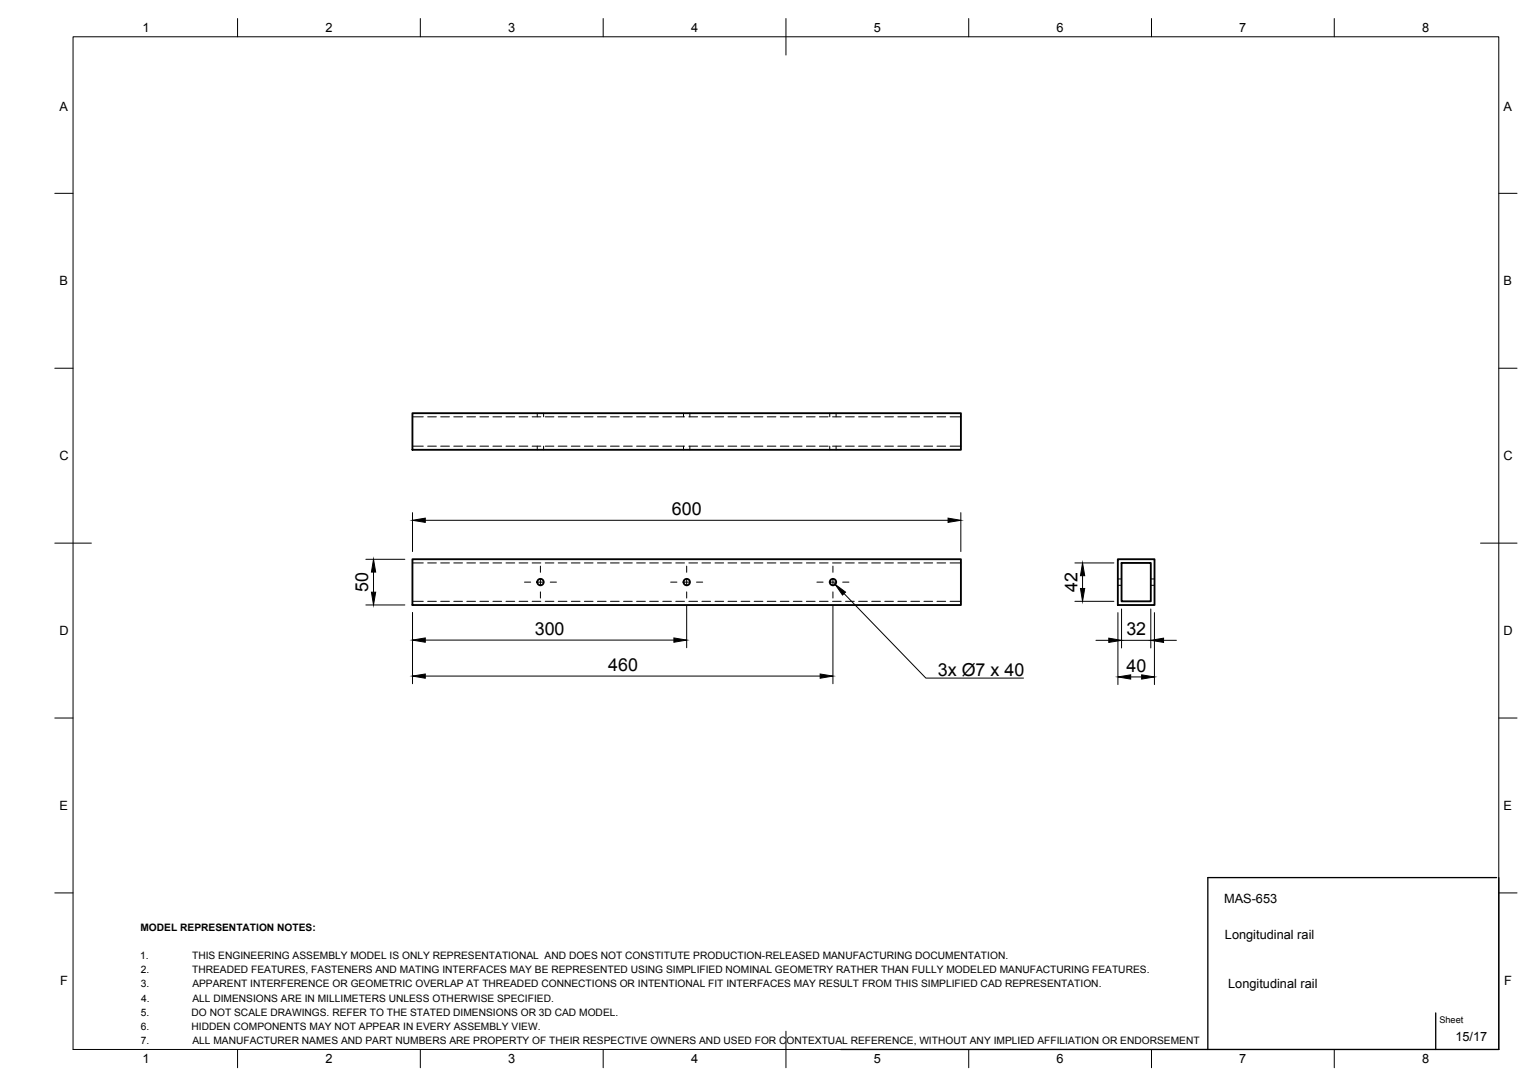
ISO-10303-21;
HEADER;
/* Generated by software containing ST-Developer
 * from STEP Tools, Inc. (www.steptools.com) 
 */

FILE_DESCRIPTION(
/* description */ ('Independent compact industrial fixture table, bolted aluminum worktop
 on connected adjustable support base. Whole-mm nominal dimensions. No
 load rating assigned.'),
/* implementation_level */ '2;1');

FILE_NAME(
/* name */ 'Longitudinal rail.step',
/* time_stamp */ '2026-11-07T17:47:58-08:00',
/* author */ (''),
/* organization */ (''),
/* preprocessor_version */ 'ST-DEVELOPER v20.2',
/* originating_system */ 'Autodesk Translation Framework v15.17.0.0',
/* authorisation */ '');

FILE_SCHEMA (('AUTOMOTIVE_DESIGN { 1 0 10303 214 3 1 1 }'));
ENDSEC;

DATA;
#10=MECHANICAL_DESIGN_GEOMETRIC_PRESENTATION_REPRESENTATION('',(#2250),#97475);
#2212=SHAPE_REPRESENTATION_RELATIONSHIP('SRR','None',#97605,#2231);
#2231=ADVANCED_BREP_SHAPE_REPRESENTATION('',(#2269),#97455);
#2250=STYLED_ITEM('',(#97718),#2269);
#2269=MANIFOLD_SOLID_BREP('Body1',#21811);
#2288=FACE_BOUND('',#3699,.T.);
#2289=FACE_BOUND('',#3700,.T.);
#2290=FACE_BOUND('',#3701,.T.);
#2291=FACE_BOUND('',#3704,.T.);
#2292=FACE_BOUND('',#3705,.T.);
#2293=FACE_BOUND('',#3706,.T.);
#2294=FACE_BOUND('',#3709,.T.);
#2295=FACE_BOUND('',#3710,.T.);
#2296=FACE_BOUND('',#3711,.T.);
#2297=FACE_BOUND('',#3714,.T.);
#2298=FACE_BOUND('',#3715,.T.);
#2299=FACE_BOUND('',#3716,.T.);
#2300=FACE_BOUND('',#3718,.T.);
#2301=FACE_BOUND('',#3720,.T.);
#2379=PLANE('',#22061);
#2380=PLANE('',#22062);
#2381=PLANE('',#22063);
#2382=PLANE('',#22064);
#2383=PLANE('',#22065);
#2384=PLANE('',#22066);
#2385=PLANE('',#22067);
#2386=PLANE('',#22068);
#2387=PLANE('',#22069);
#2388=PLANE('',#22070);
#2537=FACE_OUTER_BOUND('',#3691,.T.);
#2538=FACE_OUTER_BOUND('',#3692,.T.);
#2539=FACE_OUTER_BOUND('',#3693,.T.);
#2540=FACE_OUTER_BOUND('',#3694,.T.);
#2541=FACE_OUTER_BOUND('',#3695,.T.);
#2542=FACE_OUTER_BOUND('',#3696,.T.);
#2543=FACE_OUTER_BOUND('',#3697,.T.);
#2544=FACE_OUTER_BOUND('',#3698,.T.);
#2545=FACE_OUTER_BOUND('',#3702,.T.);
#2546=FACE_OUTER_BOUND('',#3703,.T.);
#2547=FACE_OUTER_BOUND('',#3707,.T.);
#2548=FACE_OUTER_BOUND('',#3708,.T.);
#2549=FACE_OUTER_BOUND('',#3712,.T.);
#2550=FACE_OUTER_BOUND('',#3713,.T.);
#2551=FACE_OUTER_BOUND('',#3717,.T.);
#2552=FACE_OUTER_BOUND('',#3719,.T.);
#3691=EDGE_LOOP('',(#13112,#13113,#13114,#13115));
#3692=EDGE_LOOP('',(#13116,#13117,#13118,#13119));
#3693=EDGE_LOOP('',(#13120,#13121,#13122,#13123));
#3694=EDGE_LOOP('',(#13124,#13125,#13126,#13127));
#3695=EDGE_LOOP('',(#13128,#13129,#13130,#13131));
#3696=EDGE_LOOP('',(#13132,#13133,#13134,#13135));
#3697=EDGE_LOOP('',(#13136,#13137,#13138,#13139));
#3698=EDGE_LOOP('',(#13140,#13141,#13142,#13143));
#3699=EDGE_LOOP('',(#13144));
#3700=EDGE_LOOP('',(#13145));
#3701=EDGE_LOOP('',(#13146));
#3702=EDGE_LOOP('',(#13147,#13148,#13149,#13150));
#3703=EDGE_LOOP('',(#13151,#13152,#13153,#13154));
#3704=EDGE_LOOP('',(#13155));
#3705=EDGE_LOOP('',(#13156));
#3706=EDGE_LOOP('',(#13157));
#3707=EDGE_LOOP('',(#13158,#13159,#13160,#13161));
#3708=EDGE_LOOP('',(#13162,#13163,#13164,#13165));
#3709=EDGE_LOOP('',(#13166));
#3710=EDGE_LOOP('',(#13167));
#3711=EDGE_LOOP('',(#13168));
#3712=EDGE_LOOP('',(#13169,#13170,#13171,#13172));
#3713=EDGE_LOOP('',(#13173,#13174,#13175,#13176));
#3714=EDGE_LOOP('',(#13177));
#3715=EDGE_LOOP('',(#13178));
#3716=EDGE_LOOP('',(#13179));
#3717=EDGE_LOOP('',(#13180,#13181,#13182,#13183));
#3718=EDGE_LOOP('',(#13184,#13185,#13186,#13187));
#3719=EDGE_LOOP('',(#13188,#13189,#13190,#13191));
#3720=EDGE_LOOP('',(#13192,#13193,#13194,#13195));
#4936=LINE('',#27647,#6150);
#4937=LINE('',#27653,#6151);
#4938=LINE('',#27659,#6152);
#4939=LINE('',#27665,#6153);
#4940=LINE('',#27671,#6154);
#4941=LINE('',#27677,#6155);
#4942=LINE('',#27682,#6156);
#4943=LINE('',#27684,#6157);
#4944=LINE('',#27686,#6158);
#4945=LINE('',#27687,#6159);
#4946=LINE('',#27690,#6160);
#4947=LINE('',#27692,#6161);
#4948=LINE('',#27693,#6162);
#4949=LINE('',#27696,#6163);
#4950=LINE('',#27698,#6164);
#4951=LINE('',#27699,#6165);
#4952=LINE('',#27701,#6166);
#4953=LINE('',#27702,#6167);
#4954=LINE('',#27706,#6168);
#4955=LINE('',#27708,#6169);
#4956=LINE('',#27710,#6170);
#4957=LINE('',#27711,#6171);
#4958=LINE('',#27714,#6172);
#4959=LINE('',#27716,#6173);
#4960=LINE('',#27717,#6174);
#4961=LINE('',#27720,#6175);
#4962=LINE('',#27722,#6176);
#4963=LINE('',#27723,#6177);
#4964=LINE('',#27725,#6178);
#4965=LINE('',#27726,#6179);
#6150=VECTOR('',#23512,3.5);
#6151=VECTOR('',#23519,3.5);
#6152=VECTOR('',#23526,3.5);
#6153=VECTOR('',#23533,3.5);
#6154=VECTOR('',#23540,3.5);
#6155=VECTOR('',#23547,3.5);
#6156=VECTOR('',#23552,10.);
#6157=VECTOR('',#23553,10.);
#6158=VECTOR('',#23554,10.);
#6159=VECTOR('',#23555,10.);
#6160=VECTOR('',#23558,10.);
#6161=VECTOR('',#23559,10.);
#6162=VECTOR('',#23560,10.);
#6163=VECTOR('',#23563,10.);
#6164=VECTOR('',#23564,10.);
#6165=VECTOR('',#23565,10.);
#6166=VECTOR('',#23568,10.);
#6167=VECTOR('',#23569,10.);
#6168=VECTOR('',#23572,10.);
#6169=VECTOR('',#23573,10.);
#6170=VECTOR('',#23574,10.);
#6171=VECTOR('',#23575,10.);
#6172=VECTOR('',#23578,10.);
#6173=VECTOR('',#23579,10.);
#6174=VECTOR('',#23580,10.);
#6175=VECTOR('',#23583,10.);
#6176=VECTOR('',#23584,10.);
#6177=VECTOR('',#23585,10.);
#6178=VECTOR('',#23588,10.);
#6179=VECTOR('',#23589,10.);
#7364=CIRCLE('',#22044,3.5);
#7365=CIRCLE('',#22045,3.5);
#7366=CIRCLE('',#22047,3.5);
#7367=CIRCLE('',#22048,3.5);
#7368=CIRCLE('',#22050,3.5);
#7369=CIRCLE('',#22051,3.5);
#7370=CIRCLE('',#22053,3.5);
#7371=CIRCLE('',#22054,3.5);
#7372=CIRCLE('',#22056,3.5);
#7373=CIRCLE('',#22057,3.5);
#7374=CIRCLE('',#22059,3.5);
#7375=CIRCLE('',#22060,3.5);
#7613=VERTEX_POINT('',#27644);
#7614=VERTEX_POINT('',#27646);
#7615=VERTEX_POINT('',#27650);
#7616=VERTEX_POINT('',#27652);
#7617=VERTEX_POINT('',#27656);
#7618=VERTEX_POINT('',#27658);
#7619=VERTEX_POINT('',#27662);
#7620=VERTEX_POINT('',#27664);
#7621=VERTEX_POINT('',#27668);
#7622=VERTEX_POINT('',#27670);
#7623=VERTEX_POINT('',#27674);
#7624=VERTEX_POINT('',#27676);
#7625=VERTEX_POINT('',#27680);
#7626=VERTEX_POINT('',#27681);
#7627=VERTEX_POINT('',#27683);
#7628=VERTEX_POINT('',#27685);
#7629=VERTEX_POINT('',#27689);
#7630=VERTEX_POINT('',#27691);
#7631=VERTEX_POINT('',#27695);
#7632=VERTEX_POINT('',#27697);
#7633=VERTEX_POINT('',#27704);
#7634=VERTEX_POINT('',#27705);
#7635=VERTEX_POINT('',#27707);
#7636=VERTEX_POINT('',#27709);
#7637=VERTEX_POINT('',#27713);
#7638=VERTEX_POINT('',#27715);
#7639=VERTEX_POINT('',#27719);
#7640=VERTEX_POINT('',#27721);
#9813=EDGE_CURVE('',#7613,#7613,#7364,.T.);
#9814=EDGE_CURVE('',#7613,#7614,#4936,.T.);
#9815=EDGE_CURVE('',#7614,#7614,#7365,.T.);
#9816=EDGE_CURVE('',#7615,#7615,#7366,.T.);
#9817=EDGE_CURVE('',#7615,#7616,#4937,.T.);
#9818=EDGE_CURVE('',#7616,#7616,#7367,.T.);
#9819=EDGE_CURVE('',#7617,#7617,#7368,.T.);
#9820=EDGE_CURVE('',#7617,#7618,#4938,.T.);
#9821=EDGE_CURVE('',#7618,#7618,#7369,.T.);
#9822=EDGE_CURVE('',#7619,#7619,#7370,.T.);
#9823=EDGE_CURVE('',#7619,#7620,#4939,.T.);
#9824=EDGE_CURVE('',#7620,#7620,#7371,.T.);
#9825=EDGE_CURVE('',#7621,#7621,#7372,.T.);
#9826=EDGE_CURVE('',#7621,#7622,#4940,.T.);
#9827=EDGE_CURVE('',#7622,#7622,#7373,.T.);
#9828=EDGE_CURVE('',#7623,#7623,#7374,.T.);
#9829=EDGE_CURVE('',#7623,#7624,#4941,.T.);
#9830=EDGE_CURVE('',#7624,#7624,#7375,.T.);
#9831=EDGE_CURVE('',#7625,#7626,#4942,.T.);
#9832=EDGE_CURVE('',#7626,#7627,#4943,.T.);
#9833=EDGE_CURVE('',#7628,#7627,#4944,.T.);
#9834=EDGE_CURVE('',#7625,#7628,#4945,.T.);
#9835=EDGE_CURVE('',#7629,#7625,#4946,.T.);
#9836=EDGE_CURVE('',#7630,#7628,#4947,.T.);
#9837=EDGE_CURVE('',#7629,#7630,#4948,.T.);
#9838=EDGE_CURVE('',#7631,#7629,#4949,.T.);
#9839=EDGE_CURVE('',#7632,#7630,#4950,.T.);
#9840=EDGE_CURVE('',#7631,#7632,#4951,.T.);
#9841=EDGE_CURVE('',#7626,#7631,#4952,.T.);
#9842=EDGE_CURVE('',#7627,#7632,#4953,.T.);
#9843=EDGE_CURVE('',#7633,#7634,#4954,.T.);
#9844=EDGE_CURVE('',#7634,#7635,#4955,.T.);
#9845=EDGE_CURVE('',#7636,#7635,#4956,.T.);
#9846=EDGE_CURVE('',#7633,#7636,#4957,.T.);
#9847=EDGE_CURVE('',#7637,#7633,#4958,.T.);
#9848=EDGE_CURVE('',#7638,#7636,#4959,.T.);
#9849=EDGE_CURVE('',#7637,#7638,#4960,.T.);
#9850=EDGE_CURVE('',#7639,#7637,#4961,.T.);
#9851=EDGE_CURVE('',#7640,#7638,#4962,.T.);
#9852=EDGE_CURVE('',#7639,#7640,#4963,.T.);
#9853=EDGE_CURVE('',#7634,#7639,#4964,.T.);
#9854=EDGE_CURVE('',#7635,#7640,#4965,.T.);
#13112=ORIENTED_EDGE('',*,*,#9813,.F.);
#13113=ORIENTED_EDGE('',*,*,#9814,.T.);
#13114=ORIENTED_EDGE('',*,*,#9815,.F.);
#13115=ORIENTED_EDGE('',*,*,#9814,.F.);
#13116=ORIENTED_EDGE('',*,*,#9816,.F.);
#13117=ORIENTED_EDGE('',*,*,#9817,.T.);
#13118=ORIENTED_EDGE('',*,*,#9818,.F.);
#13119=ORIENTED_EDGE('',*,*,#9817,.F.);
#13120=ORIENTED_EDGE('',*,*,#9819,.F.);
#13121=ORIENTED_EDGE('',*,*,#9820,.T.);
#13122=ORIENTED_EDGE('',*,*,#9821,.F.);
#13123=ORIENTED_EDGE('',*,*,#9820,.F.);
#13124=ORIENTED_EDGE('',*,*,#9822,.F.);
#13125=ORIENTED_EDGE('',*,*,#9823,.T.);
#13126=ORIENTED_EDGE('',*,*,#9824,.F.);
#13127=ORIENTED_EDGE('',*,*,#9823,.F.);
#13128=ORIENTED_EDGE('',*,*,#9825,.F.);
#13129=ORIENTED_EDGE('',*,*,#9826,.T.);
#13130=ORIENTED_EDGE('',*,*,#9827,.F.);
#13131=ORIENTED_EDGE('',*,*,#9826,.F.);
#13132=ORIENTED_EDGE('',*,*,#9828,.F.);
#13133=ORIENTED_EDGE('',*,*,#9829,.T.);
#13134=ORIENTED_EDGE('',*,*,#9830,.F.);
#13135=ORIENTED_EDGE('',*,*,#9829,.F.);
#13136=ORIENTED_EDGE('',*,*,#9831,.T.);
#13137=ORIENTED_EDGE('',*,*,#9832,.T.);
#13138=ORIENTED_EDGE('',*,*,#9833,.F.);
#13139=ORIENTED_EDGE('',*,*,#9834,.F.);
#13140=ORIENTED_EDGE('',*,*,#9835,.T.);
#13141=ORIENTED_EDGE('',*,*,#9834,.T.);
#13142=ORIENTED_EDGE('',*,*,#9836,.F.);
#13143=ORIENTED_EDGE('',*,*,#9837,.F.);
#13144=ORIENTED_EDGE('',*,*,#9818,.T.);
#13145=ORIENTED_EDGE('',*,*,#9824,.T.);
#13146=ORIENTED_EDGE('',*,*,#9830,.T.);
#13147=ORIENTED_EDGE('',*,*,#9838,.T.);
#13148=ORIENTED_EDGE('',*,*,#9837,.T.);
#13149=ORIENTED_EDGE('',*,*,#9839,.F.);
#13150=ORIENTED_EDGE('',*,*,#9840,.F.);
#13151=ORIENTED_EDGE('',*,*,#9841,.T.);
#13152=ORIENTED_EDGE('',*,*,#9840,.T.);
#13153=ORIENTED_EDGE('',*,*,#9842,.F.);
#13154=ORIENTED_EDGE('',*,*,#9832,.F.);
#13155=ORIENTED_EDGE('',*,*,#9813,.T.);
#13156=ORIENTED_EDGE('',*,*,#9819,.T.);
#13157=ORIENTED_EDGE('',*,*,#9825,.T.);
#13158=ORIENTED_EDGE('',*,*,#9843,.T.);
#13159=ORIENTED_EDGE('',*,*,#9844,.T.);
#13160=ORIENTED_EDGE('',*,*,#9845,.F.);
#13161=ORIENTED_EDGE('',*,*,#9846,.F.);
#13162=ORIENTED_EDGE('',*,*,#9847,.T.);
#13163=ORIENTED_EDGE('',*,*,#9846,.T.);
#13164=ORIENTED_EDGE('',*,*,#9848,.F.);
#13165=ORIENTED_EDGE('',*,*,#9849,.F.);
#13166=ORIENTED_EDGE('',*,*,#9816,.T.);
#13167=ORIENTED_EDGE('',*,*,#9822,.T.);
#13168=ORIENTED_EDGE('',*,*,#9828,.T.);
#13169=ORIENTED_EDGE('',*,*,#9850,.T.);
#13170=ORIENTED_EDGE('',*,*,#9849,.T.);
#13171=ORIENTED_EDGE('',*,*,#9851,.F.);
#13172=ORIENTED_EDGE('',*,*,#9852,.F.);
#13173=ORIENTED_EDGE('',*,*,#9853,.T.);
#13174=ORIENTED_EDGE('',*,*,#9852,.T.);
#13175=ORIENTED_EDGE('',*,*,#9854,.F.);
#13176=ORIENTED_EDGE('',*,*,#9844,.F.);
#13177=ORIENTED_EDGE('',*,*,#9815,.T.);
#13178=ORIENTED_EDGE('',*,*,#9821,.T.);
#13179=ORIENTED_EDGE('',*,*,#9827,.T.);
#13180=ORIENTED_EDGE('',*,*,#9854,.T.);
#13181=ORIENTED_EDGE('',*,*,#9851,.T.);
#13182=ORIENTED_EDGE('',*,*,#9848,.T.);
#13183=ORIENTED_EDGE('',*,*,#9845,.T.);
#13184=ORIENTED_EDGE('',*,*,#9842,.T.);
#13185=ORIENTED_EDGE('',*,*,#9839,.T.);
#13186=ORIENTED_EDGE('',*,*,#9836,.T.);
#13187=ORIENTED_EDGE('',*,*,#9833,.T.);
#13188=ORIENTED_EDGE('',*,*,#9853,.F.);
#13189=ORIENTED_EDGE('',*,*,#9843,.F.);
#13190=ORIENTED_EDGE('',*,*,#9847,.F.);
#13191=ORIENTED_EDGE('',*,*,#9850,.F.);
#13192=ORIENTED_EDGE('',*,*,#9841,.F.);
#13193=ORIENTED_EDGE('',*,*,#9831,.F.);
#13194=ORIENTED_EDGE('',*,*,#9835,.F.);
#13195=ORIENTED_EDGE('',*,*,#9838,.F.);
#19710=CYLINDRICAL_SURFACE('',#22043,3.5);
#19711=CYLINDRICAL_SURFACE('',#22046,3.5);
#19712=CYLINDRICAL_SURFACE('',#22049,3.5);
#19713=CYLINDRICAL_SURFACE('',#22052,3.5);
#19714=CYLINDRICAL_SURFACE('',#22055,3.5);
#19715=CYLINDRICAL_SURFACE('',#22058,3.5);
#20657=ADVANCED_FACE('',(#2537),#19710,.F.);
#20658=ADVANCED_FACE('',(#2538),#19711,.F.);
#20659=ADVANCED_FACE('',(#2539),#19712,.F.);
#20660=ADVANCED_FACE('',(#2540),#19713,.F.);
#20661=ADVANCED_FACE('',(#2541),#19714,.F.);
#20662=ADVANCED_FACE('',(#2542),#19715,.F.);
#20663=ADVANCED_FACE('',(#2543),#2379,.T.);
#20664=ADVANCED_FACE('',(#2544,#2288,#2289,#2290),#2380,.T.);
#20665=ADVANCED_FACE('',(#2545),#2381,.T.);
#20666=ADVANCED_FACE('',(#2546,#2291,#2292,#2293),#2382,.T.);
#20667=ADVANCED_FACE('',(#2547),#2383,.T.);
#20668=ADVANCED_FACE('',(#2548,#2294,#2295,#2296),#2384,.T.);
#20669=ADVANCED_FACE('',(#2549),#2385,.T.);
#20670=ADVANCED_FACE('',(#2550,#2297,#2298,#2299),#2386,.T.);
#20671=ADVANCED_FACE('',(#2551,#2300),#2387,.T.);
#20672=ADVANCED_FACE('',(#2552,#2301),#2388,.F.);
#21811=CLOSED_SHELL('',(#20657,#20658,#20659,#20660,#20661,#20662,#20663,
#20664,#20665,#20666,#20667,#20668,#20669,#20670,#20671,#20672));
#22042=AXIS2_PLACEMENT_3D('',#27642,#23506,#23507);
#22043=AXIS2_PLACEMENT_3D('',#27643,#23508,#23509);
#22044=AXIS2_PLACEMENT_3D('',#27645,#23510,#23511);
#22045=AXIS2_PLACEMENT_3D('',#27648,#23513,#23514);
#22046=AXIS2_PLACEMENT_3D('',#27649,#23515,#23516);
#22047=AXIS2_PLACEMENT_3D('',#27651,#23517,#23518);
#22048=AXIS2_PLACEMENT_3D('',#27654,#23520,#23521);
#22049=AXIS2_PLACEMENT_3D('',#27655,#23522,#23523);
#22050=AXIS2_PLACEMENT_3D('',#27657,#23524,#23525);
#22051=AXIS2_PLACEMENT_3D('',#27660,#23527,#23528);
#22052=AXIS2_PLACEMENT_3D('',#27661,#23529,#23530);
#22053=AXIS2_PLACEMENT_3D('',#27663,#23531,#23532);
#22054=AXIS2_PLACEMENT_3D('',#27666,#23534,#23535);
#22055=AXIS2_PLACEMENT_3D('',#27667,#23536,#23537);
#22056=AXIS2_PLACEMENT_3D('',#27669,#23538,#23539);
#22057=AXIS2_PLACEMENT_3D('',#27672,#23541,#23542);
#22058=AXIS2_PLACEMENT_3D('',#27673,#23543,#23544);
#22059=AXIS2_PLACEMENT_3D('',#27675,#23545,#23546);
#22060=AXIS2_PLACEMENT_3D('',#27678,#23548,#23549);
#22061=AXIS2_PLACEMENT_3D('',#27679,#23550,#23551);
#22062=AXIS2_PLACEMENT_3D('',#27688,#23556,#23557);
#22063=AXIS2_PLACEMENT_3D('',#27694,#23561,#23562);
#22064=AXIS2_PLACEMENT_3D('',#27700,#23566,#23567);
#22065=AXIS2_PLACEMENT_3D('',#27703,#23570,#23571);
#22066=AXIS2_PLACEMENT_3D('',#27712,#23576,#23577);
#22067=AXIS2_PLACEMENT_3D('',#27718,#23581,#23582);
#22068=AXIS2_PLACEMENT_3D('',#27724,#23586,#23587);
#22069=AXIS2_PLACEMENT_3D('',#27727,#23590,#23591);
#22070=AXIS2_PLACEMENT_3D('',#27728,#23592,#23593);
#23506=DIRECTION('axis',(0.,0.,1.));
#23507=DIRECTION('refdir',(1.,0.,0.));
#23508=DIRECTION('center_axis',(-1.,0.,0.));
#23509=DIRECTION('ref_axis',(0.,1.,0.));
#23510=DIRECTION('center_axis',(-1.,0.,0.));
#23511=DIRECTION('ref_axis',(0.,1.,0.));
#23512=DIRECTION('',(-1.,0.,0.));
#23513=DIRECTION('center_axis',(1.,0.,0.));
#23514=DIRECTION('ref_axis',(0.,1.,0.));
#23515=DIRECTION('center_axis',(-1.,0.,0.));
#23516=DIRECTION('ref_axis',(0.,1.,0.));
#23517=DIRECTION('center_axis',(-1.,0.,0.));
#23518=DIRECTION('ref_axis',(0.,1.,0.));
#23519=DIRECTION('',(-1.,0.,0.));
#23520=DIRECTION('center_axis',(1.,0.,0.));
#23521=DIRECTION('ref_axis',(0.,1.,0.));
#23522=DIRECTION('center_axis',(-1.,0.,0.));
#23523=DIRECTION('ref_axis',(0.,1.,0.));
#23524=DIRECTION('center_axis',(-1.,0.,0.));
#23525=DIRECTION('ref_axis',(0.,1.,0.));
#23526=DIRECTION('',(-1.,0.,0.));
#23527=DIRECTION('center_axis',(1.,0.,0.));
#23528=DIRECTION('ref_axis',(0.,1.,0.));
#23529=DIRECTION('center_axis',(-1.,0.,0.));
#23530=DIRECTION('ref_axis',(0.,1.,0.));
#23531=DIRECTION('center_axis',(-1.,0.,0.));
#23532=DIRECTION('ref_axis',(0.,1.,0.));
#23533=DIRECTION('',(-1.,0.,0.));
#23534=DIRECTION('center_axis',(1.,0.,0.));
#23535=DIRECTION('ref_axis',(0.,1.,0.));
#23536=DIRECTION('center_axis',(-1.,0.,0.));
#23537=DIRECTION('ref_axis',(0.,1.,0.));
#23538=DIRECTION('center_axis',(-1.,0.,0.));
#23539=DIRECTION('ref_axis',(0.,1.,0.));
#23540=DIRECTION('',(-1.,0.,0.));
#23541=DIRECTION('center_axis',(1.,0.,0.));
#23542=DIRECTION('ref_axis',(0.,1.,0.));
#23543=DIRECTION('center_axis',(-1.,0.,0.));
#23544=DIRECTION('ref_axis',(0.,1.,0.));
#23545=DIRECTION('center_axis',(-1.,0.,0.));
#23546=DIRECTION('ref_axis',(0.,1.,0.));
#23547=DIRECTION('',(-1.,0.,0.));
#23548=DIRECTION('center_axis',(1.,0.,0.));
#23549=DIRECTION('ref_axis',(0.,1.,0.));
#23550=DIRECTION('center_axis',(0.,1.,0.));
#23551=DIRECTION('ref_axis',(-1.,0.,0.));
#23552=DIRECTION('',(-1.,0.,0.));
#23553=DIRECTION('',(0.,0.,1.));
#23554=DIRECTION('',(-1.,0.,0.));
#23555=DIRECTION('',(0.,0.,1.));
#23556=DIRECTION('center_axis',(-1.,0.,0.));
#23557=DIRECTION('ref_axis',(0.,-1.,0.));
#23558=DIRECTION('',(0.,-1.,0.));
#23559=DIRECTION('',(0.,-1.,0.));
#23560=DIRECTION('',(0.,0.,1.));
#23561=DIRECTION('center_axis',(0.,-1.,0.));
#23562=DIRECTION('ref_axis',(1.,0.,0.));
#23563=DIRECTION('',(1.,0.,0.));
#23564=DIRECTION('',(1.,0.,0.));
#23565=DIRECTION('',(0.,0.,1.));
#23566=DIRECTION('center_axis',(1.,0.,0.));
#23567=DIRECTION('ref_axis',(0.,1.,0.));
#23568=DIRECTION('',(0.,1.,0.));
#23569=DIRECTION('',(0.,1.,0.));
#23570=DIRECTION('center_axis',(0.,1.,0.));
#23571=DIRECTION('ref_axis',(-1.,0.,0.));
#23572=DIRECTION('',(-1.,0.,0.));
#23573=DIRECTION('',(0.,0.,1.));
#23574=DIRECTION('',(-1.,0.,0.));
#23575=DIRECTION('',(0.,0.,1.));
#23576=DIRECTION('center_axis',(1.,0.,0.));
#23577=DIRECTION('ref_axis',(0.,1.,0.));
#23578=DIRECTION('',(0.,1.,0.));
#23579=DIRECTION('',(0.,1.,0.));
#23580=DIRECTION('',(0.,0.,1.));
#23581=DIRECTION('center_axis',(0.,-1.,0.));
#23582=DIRECTION('ref_axis',(1.,0.,0.));
#23583=DIRECTION('',(1.,0.,0.));
#23584=DIRECTION('',(1.,0.,0.));
#23585=DIRECTION('',(0.,0.,1.));
#23586=DIRECTION('center_axis',(-1.,0.,0.));
#23587=DIRECTION('ref_axis',(0.,-1.,0.));
#23588=DIRECTION('',(0.,-1.,0.));
#23589=DIRECTION('',(0.,-1.,0.));
#23590=DIRECTION('center_axis',(0.,0.,1.));
#23591=DIRECTION('ref_axis',(1.,0.,0.));
#23592=DIRECTION('center_axis',(0.,0.,1.));
#23593=DIRECTION('ref_axis',(1.,0.,0.));
#27642=CARTESIAN_POINT('',(0.,0.,0.));
#27643=CARTESIAN_POINT('Origin',(0.,0.,300.));
#27644=CARTESIAN_POINT('',(-16.,-3.5,300.));
#27645=CARTESIAN_POINT('Origin',(-16.,0.,300.));
#27646=CARTESIAN_POINT('',(-20.,-3.5,300.));
#27647=CARTESIAN_POINT('',(0.,-3.5,300.));
#27648=CARTESIAN_POINT('Origin',(-20.,0.,300.));
#27649=CARTESIAN_POINT('Origin',(0.,0.,300.));
#27650=CARTESIAN_POINT('',(20.,-3.5,300.));
#27651=CARTESIAN_POINT('Origin',(20.,0.,300.));
#27652=CARTESIAN_POINT('',(16.,-3.5,300.));
#27653=CARTESIAN_POINT('',(0.,-3.5,300.));
#27654=CARTESIAN_POINT('Origin',(16.,0.,300.));
#27655=CARTESIAN_POINT('Origin',(0.,0.,140.));
#27656=CARTESIAN_POINT('',(-16.,-3.5,140.));
#27657=CARTESIAN_POINT('Origin',(-16.,0.,140.));
#27658=CARTESIAN_POINT('',(-20.,-3.5,140.));
#27659=CARTESIAN_POINT('',(0.,-3.5,140.));
#27660=CARTESIAN_POINT('Origin',(-20.,0.,140.));
#27661=CARTESIAN_POINT('Origin',(0.,0.,140.));
#27662=CARTESIAN_POINT('',(20.,-3.5,140.));
#27663=CARTESIAN_POINT('Origin',(20.,0.,140.));
#27664=CARTESIAN_POINT('',(16.,-3.5,140.));
#27665=CARTESIAN_POINT('',(0.,-3.5,140.));
#27666=CARTESIAN_POINT('Origin',(16.,0.,140.));
#27667=CARTESIAN_POINT('Origin',(0.,0.,460.));
#27668=CARTESIAN_POINT('',(-16.,-3.5,460.));
#27669=CARTESIAN_POINT('Origin',(-16.,0.,460.));
#27670=CARTESIAN_POINT('',(-20.,-3.5,460.));
#27671=CARTESIAN_POINT('',(0.,-3.5,460.));
#27672=CARTESIAN_POINT('Origin',(-20.,0.,460.));
#27673=CARTESIAN_POINT('Origin',(0.,0.,460.));
#27674=CARTESIAN_POINT('',(20.,-3.5,460.));
#27675=CARTESIAN_POINT('Origin',(20.,0.,460.));
#27676=CARTESIAN_POINT('',(16.,-3.5,460.));
#27677=CARTESIAN_POINT('',(0.,-3.5,460.));
#27678=CARTESIAN_POINT('Origin',(16.,0.,460.));
#27679=CARTESIAN_POINT('Origin',(16.,-21.,0.));
#27680=CARTESIAN_POINT('',(16.,-21.,0.));
#27681=CARTESIAN_POINT('',(-16.,-21.,0.));
#27682=CARTESIAN_POINT('',(-16.,-21.,0.));
#27683=CARTESIAN_POINT('',(-16.,-21.,600.));
#27684=CARTESIAN_POINT('',(-16.,-21.,0.));
#27685=CARTESIAN_POINT('',(16.,-21.,600.));
#27686=CARTESIAN_POINT('',(-16.,-21.,600.));
#27687=CARTESIAN_POINT('',(16.,-21.,0.));
#27688=CARTESIAN_POINT('Origin',(16.,21.,0.));
#27689=CARTESIAN_POINT('',(16.,21.,0.));
#27690=CARTESIAN_POINT('',(16.,-21.,0.));
#27691=CARTESIAN_POINT('',(16.,21.,600.));
#27692=CARTESIAN_POINT('',(16.,-21.,600.));
#27693=CARTESIAN_POINT('',(16.,21.,0.));
#27694=CARTESIAN_POINT('Origin',(-16.,21.,0.));
#27695=CARTESIAN_POINT('',(-16.,21.,0.));
#27696=CARTESIAN_POINT('',(16.,21.,0.));
#27697=CARTESIAN_POINT('',(-16.,21.,600.));
#27698=CARTESIAN_POINT('',(16.,21.,600.));
#27699=CARTESIAN_POINT('',(-16.,21.,0.));
#27700=CARTESIAN_POINT('Origin',(-16.,-21.,0.));
#27701=CARTESIAN_POINT('',(-16.,21.,0.));
#27702=CARTESIAN_POINT('',(-16.,21.,600.));
#27703=CARTESIAN_POINT('Origin',(20.,25.,0.));
#27704=CARTESIAN_POINT('',(20.,25.,0.));
#27705=CARTESIAN_POINT('',(-20.,25.,0.));
#27706=CARTESIAN_POINT('',(20.,25.,0.));
#27707=CARTESIAN_POINT('',(-20.,25.,600.));
#27708=CARTESIAN_POINT('',(-20.,25.,0.));
#27709=CARTESIAN_POINT('',(20.,25.,600.));
#27710=CARTESIAN_POINT('',(20.,25.,600.));
#27711=CARTESIAN_POINT('',(20.,25.,0.));
#27712=CARTESIAN_POINT('Origin',(20.,-25.,0.));
#27713=CARTESIAN_POINT('',(20.,-25.,0.));
#27714=CARTESIAN_POINT('',(20.,-25.,0.));
#27715=CARTESIAN_POINT('',(20.,-25.,600.));
#27716=CARTESIAN_POINT('',(20.,-25.,600.));
#27717=CARTESIAN_POINT('',(20.,-25.,0.));
#27718=CARTESIAN_POINT('Origin',(-20.,-25.,0.));
#27719=CARTESIAN_POINT('',(-20.,-25.,0.));
#27720=CARTESIAN_POINT('',(-20.,-25.,0.));
#27721=CARTESIAN_POINT('',(-20.,-25.,600.));
#27722=CARTESIAN_POINT('',(-20.,-25.,600.));
#27723=CARTESIAN_POINT('',(-20.,-25.,0.));
#27724=CARTESIAN_POINT('Origin',(-20.,25.,0.));
#27725=CARTESIAN_POINT('',(-20.,25.,0.));
#27726=CARTESIAN_POINT('',(-20.,25.,600.));
#27727=CARTESIAN_POINT('Origin',(0.,0.,600.));
#27728=CARTESIAN_POINT('Origin',(0.,0.,0.));
#97432=UNCERTAINTY_MEASURE_WITH_UNIT(LENGTH_MEASURE(0.01),#97476,
'DISTANCE_ACCURACY_VALUE',
'Maximum model space distance between geometric entities at asserted c
onnectivities');
#97452=UNCERTAINTY_MEASURE_WITH_UNIT(LENGTH_MEASURE(0.01),#97476,
'DISTANCE_ACCURACY_VALUE',
'Maximum model space distance between geometric entities at asserted c
onnectivities');
#97455=(
GEOMETRIC_REPRESENTATION_CONTEXT(3)
GLOBAL_UNCERTAINTY_ASSIGNED_CONTEXT((#97432))
GLOBAL_UNIT_ASSIGNED_CONTEXT((#97476,#97478,#97479))
REPRESENTATION_CONTEXT('','3D')
);
#97475=(
GEOMETRIC_REPRESENTATION_CONTEXT(3)
GLOBAL_UNCERTAINTY_ASSIGNED_CONTEXT((#97452))
GLOBAL_UNIT_ASSIGNED_CONTEXT((#97476,#97478,#97479))
REPRESENTATION_CONTEXT('','3D')
);
#97476=(
LENGTH_UNIT()
NAMED_UNIT(*)
SI_UNIT(.MILLI.,.METRE.)
);
#97478=(
NAMED_UNIT(*)
PLANE_ANGLE_UNIT()
SI_UNIT($,.RADIAN.)
);
#97479=(
NAMED_UNIT(*)
SI_UNIT($,.STERADIAN.)
SOLID_ANGLE_UNIT()
);
#97482=SHAPE_DEFINITION_REPRESENTATION(#97504,#97605);
#97504=PRODUCT_DEFINITION_SHAPE('',$,#97628);
#97605=SHAPE_REPRESENTATION('',(#22042),#97455);
#97625=PRODUCT_DEFINITION_CONTEXT('part definition',#97693,'design');
#97628=PRODUCT_DEFINITION('Longitudinal rail','Longitudinal rail',#97650,
#97625);
#97650=PRODUCT_DEFINITION_FORMATION('',$,#97697);
#97693=APPLICATION_CONTEXT(
'Core Data for Automotive Mechanical Design Process');
#97694=PRODUCT_CONTEXT('part definition',#97693,'mechanical');
#97697=PRODUCT('Longitudinal rail','Longitudinal rail',
'Steel rectangular hollow section, 50 x 40 mm, 4 mm wall. Square cut e
nds; weld to adjoining rails and corner plates.',(#97694));
#97718=PRESENTATION_STYLE_ASSIGNMENT((#97725));
#97725=SURFACE_STYLE_USAGE(.BOTH.,#97732);
#97732=SURFACE_SIDE_STYLE('',(#97739));
#97739=SURFACE_STYLE_FILL_AREA(#97746);
#97746=FILL_AREA_STYLE('Dark blue',(#97753));
#97753=FILL_AREA_STYLE_COLOUR('Dark blue',#97760);
#97760=COLOUR_RGB('Dark blue',0.0901960784313725,0.270588235294118,0.513725490196078);
ENDSEC;
END-ISO-10303-21;
